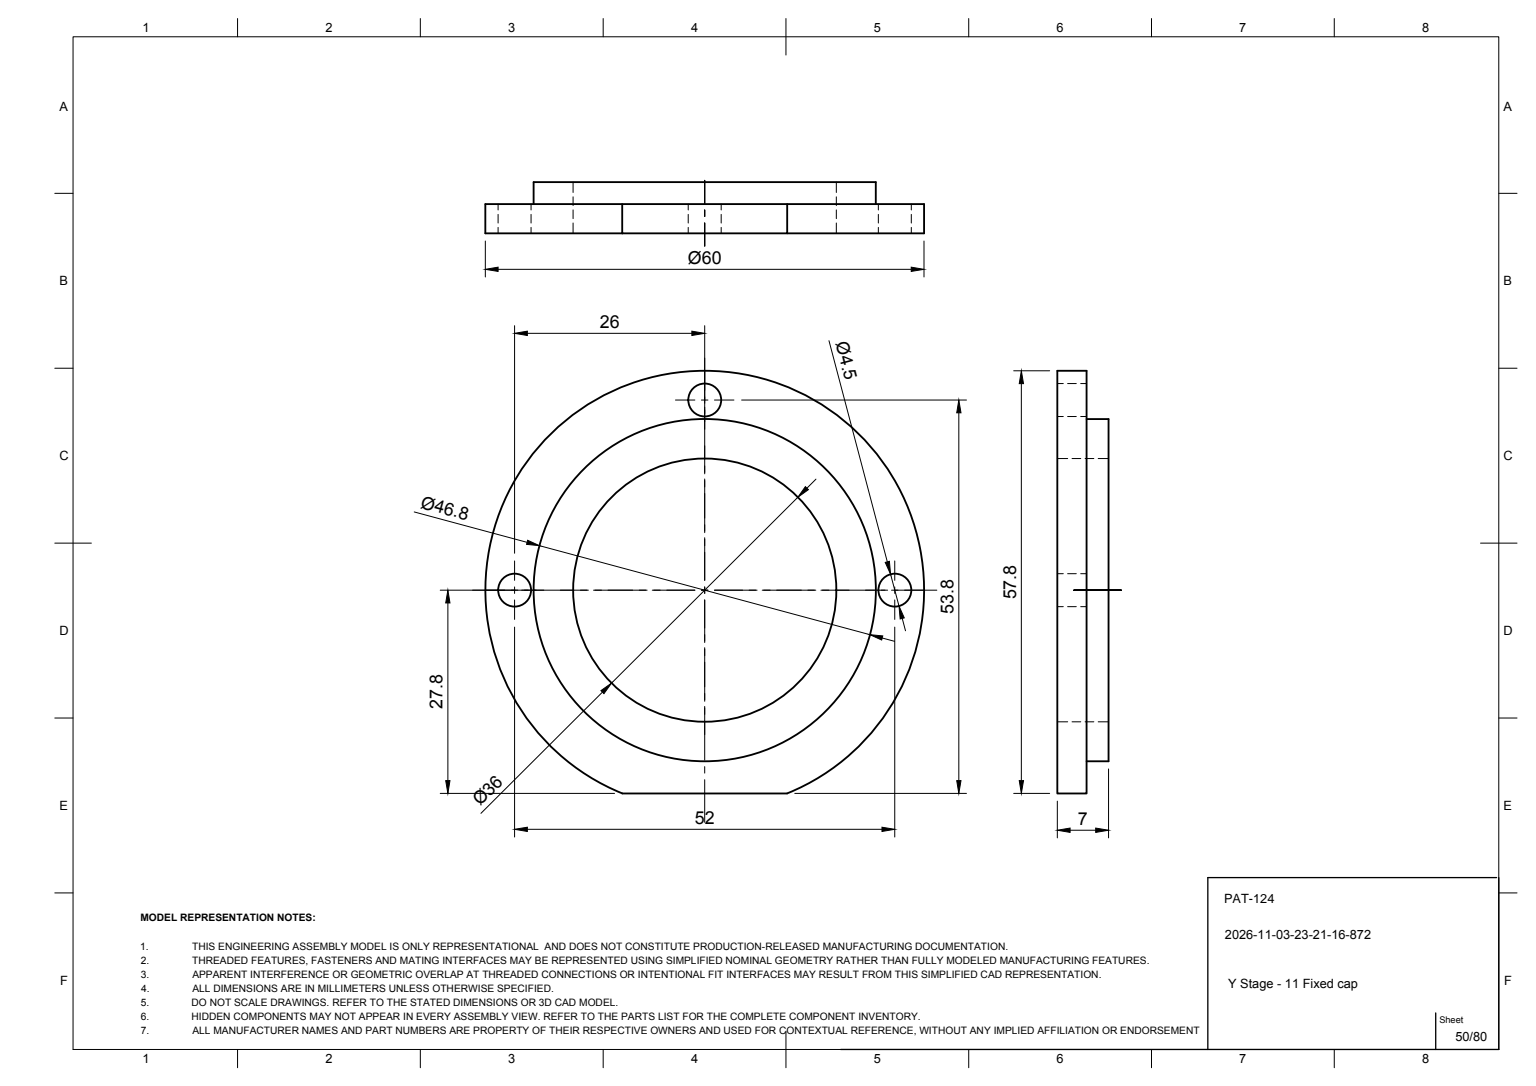
ISO-10303-21;
HEADER;
/* Generated by software containing ST-Developer
 * from STEP Tools, Inc. (www.steptools.com) 
 */

FILE_DESCRIPTION(
/* description */ ('XY cross-slide table'),
/* implementation_level */ '2;1');

FILE_NAME(
/* name */ 'Y Stage - 11 Fixed cap.step',
/* time_stamp */ '2026-10-28T03:22:46-07:00',
/* author */ (''),
/* organization */ (''),
/* preprocessor_version */ 'ST-DEVELOPER v20.2',
/* originating_system */ 'Autodesk Translation Framework v15.17.0.0',
/* authorisation */ '');

FILE_SCHEMA (('AUTOMOTIVE_DESIGN { 1 0 10303 214 3 1 1 }'));
ENDSEC;

DATA;
#10=MECHANICAL_DESIGN_GEOMETRIC_PRESENTATION_REPRESENTATION('',(#1732),#62984);
#1551=SHAPE_REPRESENTATION_RELATIONSHIP('SRR','None',#63406,#1634);
#1634=ADVANCED_BREP_SHAPE_REPRESENTATION('',(#1841),#62943);
#1732=STYLED_ITEM('',(#63926),#1841);
#1841=MANIFOLD_SOLID_BREP('Body1',#23030);
#2174=FACE_BOUND('',#5227,.T.);
#2175=FACE_BOUND('',#5228,.T.);
#2176=FACE_BOUND('',#5229,.T.);
#2177=FACE_BOUND('',#5230,.T.);
#2178=FACE_BOUND('',#5234,.T.);
#2179=FACE_BOUND('',#5237,.T.);
#2180=FACE_BOUND('',#5238,.T.);
#2181=FACE_BOUND('',#5239,.T.);
#2182=FACE_BOUND('',#5240,.T.);
#2626=PLANE('',#25446);
#2627=PLANE('',#25447);
#2628=PLANE('',#25454);
#2629=PLANE('',#25458);
#3621=FACE_OUTER_BOUND('',#5222,.T.);
#3622=FACE_OUTER_BOUND('',#5223,.T.);
#3623=FACE_OUTER_BOUND('',#5224,.T.);
#3624=FACE_OUTER_BOUND('',#5225,.T.);
#3625=FACE_OUTER_BOUND('',#5226,.T.);
#3626=FACE_OUTER_BOUND('',#5231,.T.);
#3627=FACE_OUTER_BOUND('',#5232,.T.);
#3628=FACE_OUTER_BOUND('',#5233,.T.);
#3629=FACE_OUTER_BOUND('',#5235,.T.);
#3630=FACE_OUTER_BOUND('',#5236,.T.);
#5222=EDGE_LOOP('',(#18394,#18395,#18396,#18397));
#5223=EDGE_LOOP('',(#18398,#18399,#18400,#18401));
#5224=EDGE_LOOP('',(#18402,#18403,#18404,#18405));
#5225=EDGE_LOOP('',(#18406,#18407,#18408,#18409));
#5226=EDGE_LOOP('',(#18410,#18411));
#5227=EDGE_LOOP('',(#18412));
#5228=EDGE_LOOP('',(#18413));
#5229=EDGE_LOOP('',(#18414));
#5230=EDGE_LOOP('',(#18415));
#5231=EDGE_LOOP('',(#18416,#18417,#18418,#18419));
#5232=EDGE_LOOP('',(#18420,#18421,#18422,#18423));
#5233=EDGE_LOOP('',(#18424));
#5234=EDGE_LOOP('',(#18425));
#5235=EDGE_LOOP('',(#18426,#18427,#18428,#18429));
#5236=EDGE_LOOP('',(#18430,#18431));
#5237=EDGE_LOOP('',(#18432));
#5238=EDGE_LOOP('',(#18433));
#5239=EDGE_LOOP('',(#18434));
#5240=EDGE_LOOP('',(#18435));
#6756=LINE('',#48284,#8243);
#6757=LINE('',#48290,#8244);
#6758=LINE('',#48296,#8245);
#6759=LINE('',#48301,#8246);
#6760=LINE('',#48303,#8247);
#6761=LINE('',#48305,#8248);
#6762=LINE('',#48306,#8249);
#6763=LINE('',#48315,#8250);
#6764=LINE('',#48323,#8251);
#8243=VECTOR('',#30189,0.225);
#8244=VECTOR('',#30196,0.225);
#8245=VECTOR('',#30203,0.225);
#8246=VECTOR('',#30208,1.);
#8247=VECTOR('',#30209,1.);
#8248=VECTOR('',#30210,1.);
#8249=VECTOR('',#30211,1.);
#8250=VECTOR('',#30224,2.34);
#8251=VECTOR('',#30235,1.8);
#9431=CIRCLE('',#25438,0.225);
#9432=CIRCLE('',#25439,0.225);
#9433=CIRCLE('',#25441,0.225);
#9434=CIRCLE('',#25442,0.225);
#9435=CIRCLE('',#25444,0.225);
#9436=CIRCLE('',#25445,0.225);
#9437=CIRCLE('',#25448,3.);
#9438=CIRCLE('',#25449,2.34);
#9439=CIRCLE('',#25451,3.);
#9440=CIRCLE('',#25453,2.34);
#9441=CIRCLE('',#25455,1.8);
#9442=CIRCLE('',#25457,1.8);
#10943=VERTEX_POINT('',#48281);
#10944=VERTEX_POINT('',#48283);
#10945=VERTEX_POINT('',#48287);
#10946=VERTEX_POINT('',#48289);
#10947=VERTEX_POINT('',#48293);
#10948=VERTEX_POINT('',#48295);
#10949=VERTEX_POINT('',#48299);
#10950=VERTEX_POINT('',#48300);
#10951=VERTEX_POINT('',#48302);
#10952=VERTEX_POINT('',#48304);
#10953=VERTEX_POINT('',#48309);
#10954=VERTEX_POINT('',#48314);
#10955=VERTEX_POINT('',#48318);
#10956=VERTEX_POINT('',#48321);
#13581=EDGE_CURVE('',#10943,#10943,#9431,.T.);
#13582=EDGE_CURVE('',#10943,#10944,#6756,.T.);
#13583=EDGE_CURVE('',#10944,#10944,#9432,.T.);
#13584=EDGE_CURVE('',#10945,#10945,#9433,.T.);
#13585=EDGE_CURVE('',#10945,#10946,#6757,.T.);
#13586=EDGE_CURVE('',#10946,#10946,#9434,.T.);
#13587=EDGE_CURVE('',#10947,#10947,#9435,.T.);
#13588=EDGE_CURVE('',#10947,#10948,#6758,.T.);
#13589=EDGE_CURVE('',#10948,#10948,#9436,.T.);
#13590=EDGE_CURVE('',#10949,#10950,#6759,.T.);
#13591=EDGE_CURVE('',#10951,#10949,#6760,.T.);
#13592=EDGE_CURVE('',#10952,#10951,#6761,.T.);
#13593=EDGE_CURVE('',#10950,#10952,#6762,.T.);
#13594=EDGE_CURVE('',#10951,#10949,#9437,.T.);
#13595=EDGE_CURVE('',#10953,#10953,#9438,.T.);
#13596=EDGE_CURVE('',#10952,#10950,#9439,.T.);
#13597=EDGE_CURVE('',#10953,#10954,#6763,.T.);
#13598=EDGE_CURVE('',#10954,#10954,#9440,.T.);
#13599=EDGE_CURVE('',#10955,#10955,#9441,.T.);
#13600=EDGE_CURVE('',#10956,#10956,#9442,.T.);
#13601=EDGE_CURVE('',#10956,#10955,#6764,.T.);
#18394=ORIENTED_EDGE('',*,*,#13581,.F.);
#18395=ORIENTED_EDGE('',*,*,#13582,.T.);
#18396=ORIENTED_EDGE('',*,*,#13583,.F.);
#18397=ORIENTED_EDGE('',*,*,#13582,.F.);
#18398=ORIENTED_EDGE('',*,*,#13584,.F.);
#18399=ORIENTED_EDGE('',*,*,#13585,.T.);
#18400=ORIENTED_EDGE('',*,*,#13586,.F.);
#18401=ORIENTED_EDGE('',*,*,#13585,.F.);
#18402=ORIENTED_EDGE('',*,*,#13587,.F.);
#18403=ORIENTED_EDGE('',*,*,#13588,.T.);
#18404=ORIENTED_EDGE('',*,*,#13589,.F.);
#18405=ORIENTED_EDGE('',*,*,#13588,.F.);
#18406=ORIENTED_EDGE('',*,*,#13590,.F.);
#18407=ORIENTED_EDGE('',*,*,#13591,.F.);
#18408=ORIENTED_EDGE('',*,*,#13592,.F.);
#18409=ORIENTED_EDGE('',*,*,#13593,.F.);
#18410=ORIENTED_EDGE('',*,*,#13591,.T.);
#18411=ORIENTED_EDGE('',*,*,#13594,.F.);
#18412=ORIENTED_EDGE('',*,*,#13581,.T.);
#18413=ORIENTED_EDGE('',*,*,#13584,.T.);
#18414=ORIENTED_EDGE('',*,*,#13587,.T.);
#18415=ORIENTED_EDGE('',*,*,#13595,.T.);
#18416=ORIENTED_EDGE('',*,*,#13592,.T.);
#18417=ORIENTED_EDGE('',*,*,#13594,.T.);
#18418=ORIENTED_EDGE('',*,*,#13590,.T.);
#18419=ORIENTED_EDGE('',*,*,#13596,.F.);
#18420=ORIENTED_EDGE('',*,*,#13595,.F.);
#18421=ORIENTED_EDGE('',*,*,#13597,.T.);
#18422=ORIENTED_EDGE('',*,*,#13598,.T.);
#18423=ORIENTED_EDGE('',*,*,#13597,.F.);
#18424=ORIENTED_EDGE('',*,*,#13598,.F.);
#18425=ORIENTED_EDGE('',*,*,#13599,.F.);
#18426=ORIENTED_EDGE('',*,*,#13600,.F.);
#18427=ORIENTED_EDGE('',*,*,#13601,.T.);
#18428=ORIENTED_EDGE('',*,*,#13599,.T.);
#18429=ORIENTED_EDGE('',*,*,#13601,.F.);
#18430=ORIENTED_EDGE('',*,*,#13593,.T.);
#18431=ORIENTED_EDGE('',*,*,#13596,.T.);
#18432=ORIENTED_EDGE('',*,*,#13583,.T.);
#18433=ORIENTED_EDGE('',*,*,#13586,.T.);
#18434=ORIENTED_EDGE('',*,*,#13589,.T.);
#18435=ORIENTED_EDGE('',*,*,#13600,.T.);
#21398=CYLINDRICAL_SURFACE('',#25437,0.225);
#21399=CYLINDRICAL_SURFACE('',#25440,0.225);
#21400=CYLINDRICAL_SURFACE('',#25443,0.225);
#21401=CYLINDRICAL_SURFACE('',#25450,3.);
#21402=CYLINDRICAL_SURFACE('',#25452,2.34);
#21403=CYLINDRICAL_SURFACE('',#25456,1.8);
#22402=ADVANCED_FACE('',(#3621),#21398,.F.);
#22403=ADVANCED_FACE('',(#3622),#21399,.F.);
#22404=ADVANCED_FACE('',(#3623),#21400,.F.);
#22405=ADVANCED_FACE('',(#3624),#2626,.F.);
#22406=ADVANCED_FACE('',(#3625,#2174,#2175,#2176,#2177),#2627,.F.);
#22407=ADVANCED_FACE('',(#3626),#21401,.T.);
#22408=ADVANCED_FACE('',(#3627),#21402,.T.);
#22409=ADVANCED_FACE('',(#3628,#2178),#2628,.F.);
#22410=ADVANCED_FACE('',(#3629),#21403,.F.);
#22411=ADVANCED_FACE('',(#3630,#2179,#2180,#2181,#2182),#2629,.T.);
#23030=CLOSED_SHELL('',(#22402,#22403,#22404,#22405,#22406,#22407,#22408,
#22409,#22410,#22411));
#25436=AXIS2_PLACEMENT_3D('',#48279,#30183,#30184);
#25437=AXIS2_PLACEMENT_3D('',#48280,#30185,#30186);
#25438=AXIS2_PLACEMENT_3D('',#48282,#30187,#30188);
#25439=AXIS2_PLACEMENT_3D('',#48285,#30190,#30191);
#25440=AXIS2_PLACEMENT_3D('',#48286,#30192,#30193);
#25441=AXIS2_PLACEMENT_3D('',#48288,#30194,#30195);
#25442=AXIS2_PLACEMENT_3D('',#48291,#30197,#30198);
#25443=AXIS2_PLACEMENT_3D('',#48292,#30199,#30200);
#25444=AXIS2_PLACEMENT_3D('',#48294,#30201,#30202);
#25445=AXIS2_PLACEMENT_3D('',#48297,#30204,#30205);
#25446=AXIS2_PLACEMENT_3D('',#48298,#30206,#30207);
#25447=AXIS2_PLACEMENT_3D('',#48307,#30212,#30213);
#25448=AXIS2_PLACEMENT_3D('',#48308,#30214,#30215);
#25449=AXIS2_PLACEMENT_3D('',#48310,#30216,#30217);
#25450=AXIS2_PLACEMENT_3D('',#48311,#30218,#30219);
#25451=AXIS2_PLACEMENT_3D('',#48312,#30220,#30221);
#25452=AXIS2_PLACEMENT_3D('',#48313,#30222,#30223);
#25453=AXIS2_PLACEMENT_3D('',#48316,#30225,#30226);
#25454=AXIS2_PLACEMENT_3D('',#48317,#30227,#30228);
#25455=AXIS2_PLACEMENT_3D('',#48319,#30229,#30230);
#25456=AXIS2_PLACEMENT_3D('',#48320,#30231,#30232);
#25457=AXIS2_PLACEMENT_3D('',#48322,#30233,#30234);
#25458=AXIS2_PLACEMENT_3D('',#48324,#30236,#30237);
#30183=DIRECTION('axis',(0.,0.,1.));
#30184=DIRECTION('refdir',(1.,0.,0.));
#30185=DIRECTION('center_axis',(1.,0.,0.));
#30186=DIRECTION('ref_axis',(0.,0.,-1.));
#30187=DIRECTION('center_axis',(1.,0.,0.));
#30188=DIRECTION('ref_axis',(0.,0.,-1.));
#30189=DIRECTION('',(1.,0.,0.));
#30190=DIRECTION('center_axis',(-1.,0.,0.));
#30191=DIRECTION('ref_axis',(0.,0.,-1.));
#30192=DIRECTION('center_axis',(1.,0.,0.));
#30193=DIRECTION('ref_axis',(0.,0.,-1.));
#30194=DIRECTION('center_axis',(1.,0.,0.));
#30195=DIRECTION('ref_axis',(0.,0.,-1.));
#30196=DIRECTION('',(1.,0.,0.));
#30197=DIRECTION('center_axis',(-1.,0.,0.));
#30198=DIRECTION('ref_axis',(0.,0.,-1.));
#30199=DIRECTION('center_axis',(1.,0.,0.));
#30200=DIRECTION('ref_axis',(0.,0.,-1.));
#30201=DIRECTION('center_axis',(1.,0.,0.));
#30202=DIRECTION('ref_axis',(0.,0.,-1.));
#30203=DIRECTION('',(1.,0.,0.));
#30204=DIRECTION('center_axis',(-1.,0.,0.));
#30205=DIRECTION('ref_axis',(0.,0.,-1.));
#30206=DIRECTION('center_axis',(0.,0.,1.));
#30207=DIRECTION('ref_axis',(0.,-1.,0.));
#30208=DIRECTION('',(1.,0.,0.));
#30209=DIRECTION('',(0.,-1.,0.));
#30210=DIRECTION('',(-1.,0.,0.));
#30211=DIRECTION('',(0.,1.,0.));
#30212=DIRECTION('center_axis',(1.,0.,0.));
#30213=DIRECTION('ref_axis',(0.,0.,-1.));
#30214=DIRECTION('center_axis',(1.,0.,0.));
#30215=DIRECTION('ref_axis',(0.,0.,-1.));
#30216=DIRECTION('center_axis',(1.,0.,0.));
#30217=DIRECTION('ref_axis',(0.,0.,-1.));
#30218=DIRECTION('center_axis',(1.,0.,0.));
#30219=DIRECTION('ref_axis',(0.,1.22464679914735E-16,1.));
#30220=DIRECTION('center_axis',(1.,0.,0.));
#30221=DIRECTION('ref_axis',(0.,0.,-1.));
#30222=DIRECTION('center_axis',(1.,0.,0.));
#30223=DIRECTION('ref_axis',(0.,0.,-1.));
#30224=DIRECTION('',(-1.,0.,0.));
#30225=DIRECTION('center_axis',(1.,0.,0.));
#30226=DIRECTION('ref_axis',(0.,0.,-1.));
#30227=DIRECTION('center_axis',(1.,0.,0.));
#30228=DIRECTION('ref_axis',(0.,0.,-1.));
#30229=DIRECTION('center_axis',(-1.,0.,0.));
#30230=DIRECTION('ref_axis',(0.,0.,-1.));
#30231=DIRECTION('center_axis',(1.,0.,0.));
#30232=DIRECTION('ref_axis',(0.,0.,-1.));
#30233=DIRECTION('center_axis',(-1.,0.,0.));
#30234=DIRECTION('ref_axis',(0.,0.,-1.));
#30235=DIRECTION('',(-1.,0.,0.));
#30236=DIRECTION('center_axis',(1.,0.,0.));
#30237=DIRECTION('ref_axis',(0.,0.,-1.));
#48279=CARTESIAN_POINT('',(0.,0.,0.));
#48280=CARTESIAN_POINT('Origin',(24.9,-2.6,4.));
#48281=CARTESIAN_POINT('',(25.,-2.6,4.225));
#48282=CARTESIAN_POINT('Origin',(25.,-2.6,4.));
#48283=CARTESIAN_POINT('',(25.4,-2.6,4.225));
#48284=CARTESIAN_POINT('',(24.9,-2.6,4.225));
#48285=CARTESIAN_POINT('Origin',(25.4,-2.6,4.));
#48286=CARTESIAN_POINT('Origin',(24.9,2.6,4.));
#48287=CARTESIAN_POINT('',(25.,2.6,4.225));
#48288=CARTESIAN_POINT('Origin',(25.,2.6,4.));
#48289=CARTESIAN_POINT('',(25.4,2.6,4.225));
#48290=CARTESIAN_POINT('',(24.9,2.6,4.225));
#48291=CARTESIAN_POINT('Origin',(25.4,2.6,4.));
#48292=CARTESIAN_POINT('Origin',(24.9,0.,6.6));
#48293=CARTESIAN_POINT('',(25.,-2.75545529808154E-17,6.825));
#48294=CARTESIAN_POINT('Origin',(25.,0.,6.6));
#48295=CARTESIAN_POINT('',(25.4,2.75545529808154E-17,6.825));
#48296=CARTESIAN_POINT('',(24.9,-2.75545529808154E-17,6.825));
#48297=CARTESIAN_POINT('Origin',(25.4,0.,6.6));
#48298=CARTESIAN_POINT('Origin',(24.9,3.5,1.22));
#48299=CARTESIAN_POINT('',(25.,-1.12765242872084,1.22));
#48300=CARTESIAN_POINT('',(25.4,-1.12765242872084,1.22));
#48301=CARTESIAN_POINT('',(25.,-1.12765242872084,1.22));
#48302=CARTESIAN_POINT('',(25.,1.12765242872084,1.22));
#48303=CARTESIAN_POINT('',(25.,1.75,1.22));
#48304=CARTESIAN_POINT('',(25.4,1.12765242872084,1.22));
#48305=CARTESIAN_POINT('',(25.,1.12765242872084,1.22));
#48306=CARTESIAN_POINT('',(25.4,1.75,1.22));
#48307=CARTESIAN_POINT('Origin',(25.,0.,4.));
#48308=CARTESIAN_POINT('Origin',(25.,0.,4.));
#48309=CARTESIAN_POINT('',(25.,-2.86567351000481E-16,6.34));
#48310=CARTESIAN_POINT('Origin',(25.,0.,4.));
#48311=CARTESIAN_POINT('Origin',(25.,0.,4.));
#48312=CARTESIAN_POINT('Origin',(25.4,0.,4.));
#48313=CARTESIAN_POINT('Origin',(24.7,0.,4.));
#48314=CARTESIAN_POINT('',(24.7,-2.86567351000481E-16,6.34));
#48315=CARTESIAN_POINT('',(24.7,-2.86567351000481E-16,6.34));
#48316=CARTESIAN_POINT('Origin',(24.7,0.,4.));
#48317=CARTESIAN_POINT('Origin',(24.7,0.,4.));
#48318=CARTESIAN_POINT('',(24.7,-2.20436423846524E-16,5.8));
#48319=CARTESIAN_POINT('Origin',(24.7,0.,4.));
#48320=CARTESIAN_POINT('Origin',(25.,0.,4.));
#48321=CARTESIAN_POINT('',(25.4,-2.20436423846524E-16,5.8));
#48322=CARTESIAN_POINT('Origin',(25.4,0.,4.));
#48323=CARTESIAN_POINT('',(25.,-2.20436423846524E-16,5.8));
#48324=CARTESIAN_POINT('Origin',(25.4,0.,4.));
#62844=UNCERTAINTY_MEASURE_WITH_UNIT(LENGTH_MEASURE(0.001),#62985,
'DISTANCE_ACCURACY_VALUE',
'Maximum model space distance between geometric entities at asserted c
onnectivities');
#62885=UNCERTAINTY_MEASURE_WITH_UNIT(LENGTH_MEASURE(0.001),#62985,
'DISTANCE_ACCURACY_VALUE',
'Maximum model space distance between geometric entities at asserted c
onnectivities');
#62943=(
GEOMETRIC_REPRESENTATION_CONTEXT(3)
GLOBAL_UNCERTAINTY_ASSIGNED_CONTEXT((#62844))
GLOBAL_UNIT_ASSIGNED_CONTEXT((#62985,#62987,#62988))
REPRESENTATION_CONTEXT('','3D')
);
#62984=(
GEOMETRIC_REPRESENTATION_CONTEXT(3)
GLOBAL_UNCERTAINTY_ASSIGNED_CONTEXT((#62885))
GLOBAL_UNIT_ASSIGNED_CONTEXT((#62985,#62987,#62988))
REPRESENTATION_CONTEXT('','3D')
);
#62985=(
LENGTH_UNIT()
NAMED_UNIT(*)
SI_UNIT(.CENTI.,.METRE.)
);
#62987=(
NAMED_UNIT(*)
PLANE_ANGLE_UNIT()
SI_UNIT($,.RADIAN.)
);
#62988=(
NAMED_UNIT(*)
SI_UNIT($,.STERADIAN.)
SOLID_ANGLE_UNIT()
);
#63046=SHAPE_DEFINITION_REPRESENTATION(#63224,#63406);
#63224=PRODUCT_DEFINITION_SHAPE('',$,#63505);
#63406=SHAPE_REPRESENTATION('',(#25436),#62943);
#63447=PRODUCT_DEFINITION_CONTEXT('part definition',#63743,'design');
#63505=PRODUCT_DEFINITION('Y Stage - 11 Fixed cap',
'Y Stage - 11 Fixed cap',#63603,#63447);
#63603=PRODUCT_DEFINITION_FORMATION('',$,#63802);
#63743=APPLICATION_CONTEXT(
'Core Data for Automotive Mechanical Design Process');
#63744=PRODUCT_CONTEXT('part definition',#63743,'mechanical');
#63802=PRODUCT('Y Stage - 11 Fixed cap','Y Stage - 11 Fixed cap',
'Y Stage - 11 Fixed cap',(#63744));
#63920=COLOUR_RGB('Off White',0.89,0.88,0.83);
#63921=FILL_AREA_STYLE_COLOUR('',#63920);
#63922=FILL_AREA_STYLE('',(#63921));
#63923=SURFACE_STYLE_FILL_AREA(#63922);
#63924=SURFACE_SIDE_STYLE('',(#63923));
#63925=SURFACE_STYLE_USAGE(.BOTH.,#63924);
#63926=PRESENTATION_STYLE_ASSIGNMENT((#63925));
ENDSEC;
END-ISO-10303-21;
